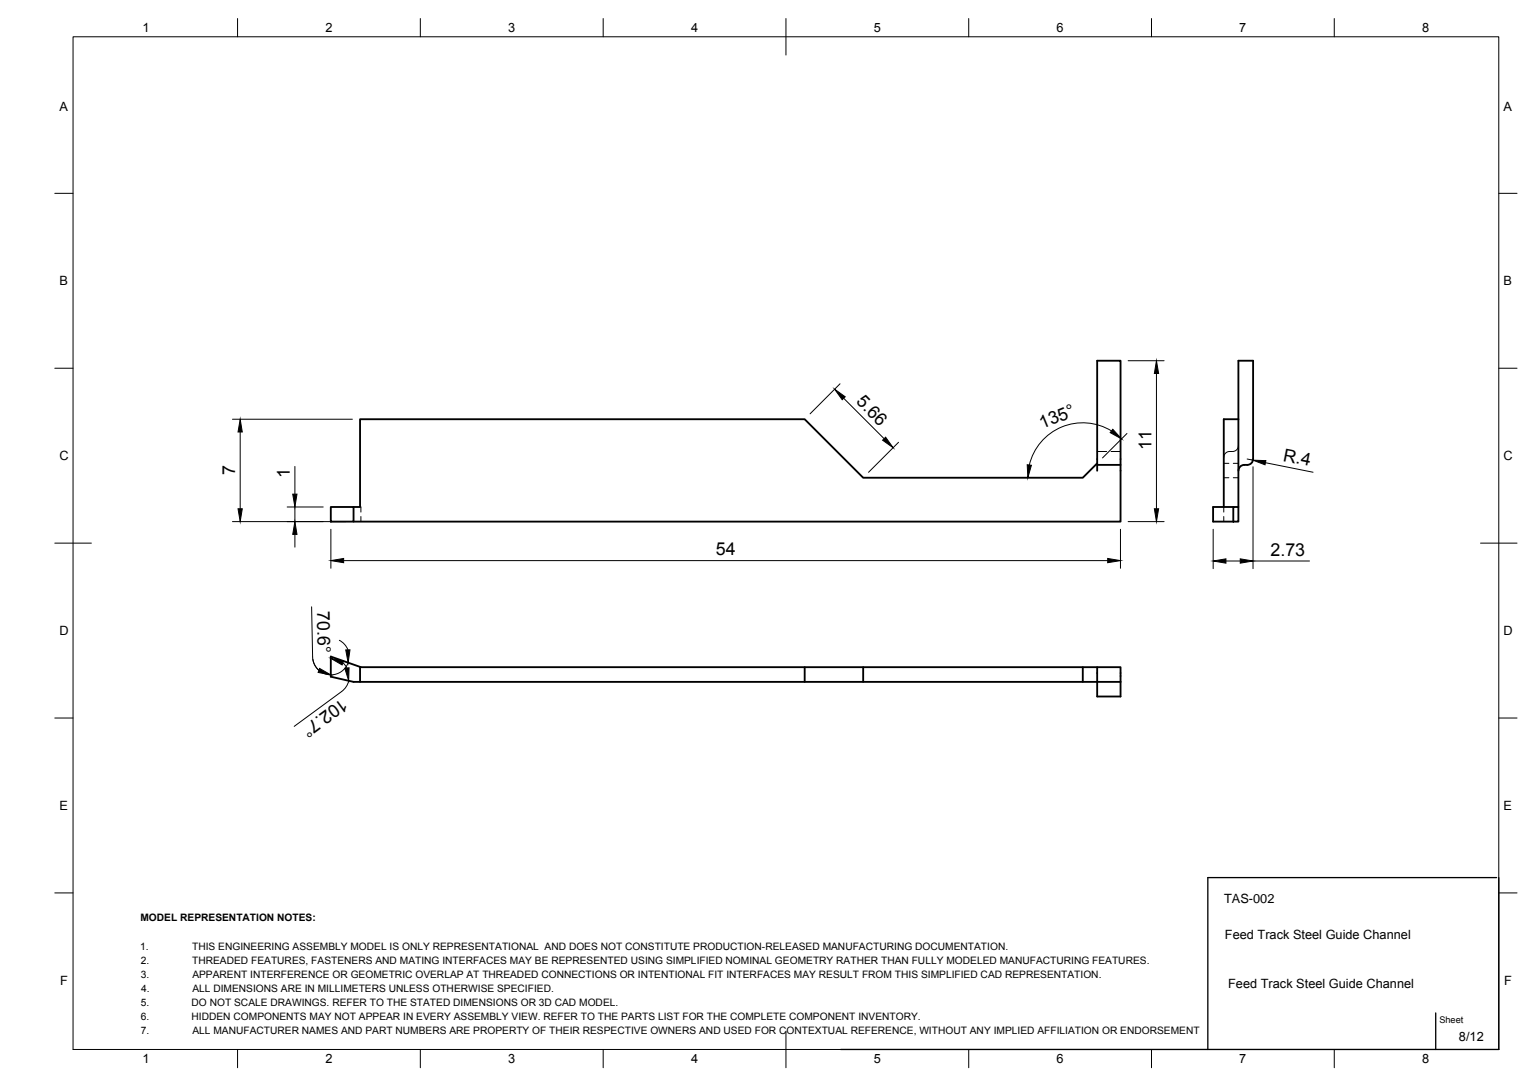
ISO-10303-21;
HEADER;
/* Generated by software containing ST-Developer
 * from STEP Tools, Inc. (www.steptools.com) 
 */

FILE_DESCRIPTION(
/* description */ ('STEP AP214'),
/* implementation_level */ '2;1');

FILE_NAME(
/* name */ 'Feed Track Steel Guide Channel.step',
/* time_stamp */ '2026-11-04T19:38:14-08:00',
/* author */ (''),
/* organization */ (''),
/* preprocessor_version */ 'ST-DEVELOPER v20.2',
/* originating_system */ 'Autodesk Translation Framework v15.17.0.0',
/* authorisation */ '');

FILE_SCHEMA (('AUTOMOTIVE_DESIGN { 1 0 10303 214 3 1 1 }'));
ENDSEC;

DATA;
#10=MECHANICAL_DESIGN_GEOMETRIC_PRESENTATION_REPRESENTATION('',(#475),#36668);
#455=SHAPE_REPRESENTATION_RELATIONSHIP('SRR','None',#36711,#465);
#465=ADVANCED_BREP_SHAPE_REPRESENTATION('',(#485),#36663);
#475=STYLED_ITEM('',(#36770),#485);
#485=MANIFOLD_SOLID_BREP('Body1',#17798);
#618=CYLINDRICAL_SURFACE('',#18758,0.399999999999998);
#619=CYLINDRICAL_SURFACE('',#18761,0.399999999999998);
#620=CYLINDRICAL_SURFACE('',#18764,0.399999999999998);
#621=CYLINDRICAL_SURFACE('',#18767,0.399999999999998);
#1353=CIRCLE('',#18759,0.399999999999998);
#1354=CIRCLE('',#18760,0.400000000000011);
#1355=CIRCLE('',#18762,0.399999999999998);
#1356=CIRCLE('',#18763,0.400000000000011);
#1357=CIRCLE('',#18765,0.400000000000011);
#1358=CIRCLE('',#18766,0.399999999999998);
#1359=CIRCLE('',#18768,0.400000000000011);
#1360=CIRCLE('',#18769,0.399999999999998);
#1973=FACE_OUTER_BOUND('',#3055,.T.);
#1974=FACE_OUTER_BOUND('',#3056,.T.);
#1975=FACE_OUTER_BOUND('',#3057,.T.);
#1976=FACE_OUTER_BOUND('',#3058,.T.);
#1977=FACE_OUTER_BOUND('',#3059,.T.);
#1978=FACE_OUTER_BOUND('',#3060,.T.);
#1979=FACE_OUTER_BOUND('',#3061,.T.);
#1980=FACE_OUTER_BOUND('',#3062,.T.);
#1981=FACE_OUTER_BOUND('',#3063,.T.);
#1982=FACE_OUTER_BOUND('',#3064,.T.);
#1983=FACE_OUTER_BOUND('',#3065,.T.);
#1984=FACE_OUTER_BOUND('',#3066,.T.);
#1985=FACE_OUTER_BOUND('',#3067,.T.);
#1986=FACE_OUTER_BOUND('',#3068,.T.);
#1987=FACE_OUTER_BOUND('',#3069,.T.);
#1988=FACE_OUTER_BOUND('',#3070,.T.);
#1989=FACE_OUTER_BOUND('',#3071,.T.);
#1990=FACE_OUTER_BOUND('',#3072,.T.);
#1991=FACE_OUTER_BOUND('',#3073,.T.);
#1992=FACE_OUTER_BOUND('',#3074,.T.);
#1993=FACE_OUTER_BOUND('',#3075,.T.);
#1994=FACE_OUTER_BOUND('',#3076,.T.);
#1995=FACE_OUTER_BOUND('',#3077,.T.);
#3055=EDGE_LOOP('',(#13714,#13715,#13716,#13717));
#3056=EDGE_LOOP('',(#13718,#13719,#13720,#13721));
#3057=EDGE_LOOP('',(#13722,#13723,#13724,#13725));
#3058=EDGE_LOOP('',(#13726,#13727,#13728,#13729));
#3059=EDGE_LOOP('',(#13730,#13731,#13732,#13733));
#3060=EDGE_LOOP('',(#13734,#13735,#13736,#13737));
#3061=EDGE_LOOP('',(#13738,#13739,#13740,#13741));
#3062=EDGE_LOOP('',(#13742,#13743,#13744,#13745));
#3063=EDGE_LOOP('',(#13746,#13747,#13748,#13749));
#3064=EDGE_LOOP('',(#13750,#13751,#13752,#13753));
#3065=EDGE_LOOP('',(#13754,#13755,#13756,#13757,#13758,#13759,#13760,#13761,
#13762,#13763,#13764));
#3066=EDGE_LOOP('',(#13765,#13766,#13767,#13768,#13769,#13770,#13771,#13772,
#13773,#13774,#13775));
#3067=EDGE_LOOP('',(#13776,#13777,#13778,#13779,#13780,#13781,#13782,#13783,
#13784,#13785,#13786,#13787));
#3068=EDGE_LOOP('',(#13788,#13789,#13790,#13791));
#3069=EDGE_LOOP('',(#13792,#13793,#13794,#13795));
#3070=EDGE_LOOP('',(#13796,#13797,#13798,#13799));
#3071=EDGE_LOOP('',(#13800,#13801,#13802,#13803));
#3072=EDGE_LOOP('',(#13804,#13805,#13806,#13807));
#3073=EDGE_LOOP('',(#13808,#13809,#13810,#13811,#13812,#13813));
#3074=EDGE_LOOP('',(#13814,#13815,#13816,#13817));
#3075=EDGE_LOOP('',(#13818,#13819,#13820,#13821,#13822,#13823,#13824,#13825,
#13826,#13827,#13828,#13829));
#3076=EDGE_LOOP('',(#13830,#13831,#13832,#13833));
#3077=EDGE_LOOP('',(#13834,#13835,#13836,#13837,#13838,#13839));
#4394=LINE('',#27429,#6104);
#4395=LINE('',#27431,#6105);
#4396=LINE('',#27433,#6106);
#4397=LINE('',#27434,#6107);
#4398=LINE('',#27438,#6108);
#4399=LINE('',#27440,#6109);
#4400=LINE('',#27442,#6110);
#4401=LINE('',#27443,#6111);
#4402=LINE('',#27449,#6112);
#4403=LINE('',#27452,#6113);
#4404=LINE('',#27458,#6114);
#4405=LINE('',#27461,#6115);
#4406=LINE('',#27467,#6116);
#4407=LINE('',#27470,#6117);
#4408=LINE('',#27476,#6118);
#4409=LINE('',#27479,#6119);
#4410=LINE('',#27482,#6120);
#4411=LINE('',#27484,#6121);
#4412=LINE('',#27485,#6122);
#4413=LINE('',#27487,#6123);
#4414=LINE('',#27488,#6124);
#4415=LINE('',#27491,#6125);
#4416=LINE('',#27493,#6126);
#4417=LINE('',#27494,#6127);
#4418=LINE('',#27496,#6128);
#4419=LINE('',#27497,#6129);
#4420=LINE('',#27500,#6130);
#4421=LINE('',#27501,#6131);
#4422=LINE('',#27503,#6132);
#4423=LINE('',#27505,#6133);
#4424=LINE('',#27507,#6134);
#4425=LINE('',#27509,#6135);
#4426=LINE('',#27511,#6136);
#4427=LINE('',#27513,#6137);
#4428=LINE('',#27514,#6138);
#4429=LINE('',#27517,#6139);
#4430=LINE('',#27518,#6140);
#4431=LINE('',#27520,#6141);
#4432=LINE('',#27522,#6142);
#4433=LINE('',#27524,#6143);
#4434=LINE('',#27526,#6144);
#4435=LINE('',#27528,#6145);
#4436=LINE('',#27530,#6146);
#4437=LINE('',#27531,#6147);
#4438=LINE('',#27533,#6148);
#4439=LINE('',#27534,#6149);
#4440=LINE('',#27536,#6150);
#4441=LINE('',#27538,#6151);
#4442=LINE('',#27540,#6152);
#4443=LINE('',#27542,#6153);
#4444=LINE('',#27544,#6154);
#4445=LINE('',#27546,#6155);
#4446=LINE('',#27548,#6156);
#4447=LINE('',#27550,#6157);
#4448=LINE('',#27551,#6158);
#6104=VECTOR('',#21930,1000.);
#6105=VECTOR('',#21931,1000.);
#6106=VECTOR('',#21932,1000.);
#6107=VECTOR('',#21933,1000.);
#6108=VECTOR('',#21936,1000.);
#6109=VECTOR('',#21937,1000.);
#6110=VECTOR('',#21938,1000.);
#6111=VECTOR('',#21939,1000.);
#6112=VECTOR('',#21944,1000.);
#6113=VECTOR('',#21947,1000.);
#6114=VECTOR('',#21952,1000.);
#6115=VECTOR('',#21955,1000.);
#6116=VECTOR('',#21960,1000.);
#6117=VECTOR('',#21963,1000.);
#6118=VECTOR('',#21968,1000.);
#6119=VECTOR('',#21971,1000.);
#6120=VECTOR('',#21974,1000.);
#6121=VECTOR('',#21975,1000.);
#6122=VECTOR('',#21976,1000.);
#6123=VECTOR('',#21979,1000.);
#6124=VECTOR('',#21980,1000.);
#6125=VECTOR('',#21983,1000.);
#6126=VECTOR('',#21984,1000.);
#6127=VECTOR('',#21985,1000.);
#6128=VECTOR('',#21988,1000.);
#6129=VECTOR('',#21989,1000.);
#6130=VECTOR('',#21992,1000.);
#6131=VECTOR('',#21993,1000.);
#6132=VECTOR('',#21994,1000.);
#6133=VECTOR('',#21995,1000.);
#6134=VECTOR('',#21996,1000.);
#6135=VECTOR('',#21997,1000.);
#6136=VECTOR('',#21998,1000.);
#6137=VECTOR('',#21999,1000.);
#6138=VECTOR('',#22000,1000.);
#6139=VECTOR('',#22003,1000.);
#6140=VECTOR('',#22004,1000.);
#6141=VECTOR('',#22005,1000.);
#6142=VECTOR('',#22006,1000.);
#6143=VECTOR('',#22007,1000.);
#6144=VECTOR('',#22008,1000.);
#6145=VECTOR('',#22009,1000.);
#6146=VECTOR('',#22010,1000.);
#6147=VECTOR('',#22011,1000.);
#6148=VECTOR('',#22014,1000.);
#6149=VECTOR('',#22015,1000.);
#6150=VECTOR('',#22018,1000.);
#6151=VECTOR('',#22021,1000.);
#6152=VECTOR('',#22024,1000.);
#6153=VECTOR('',#22027,1000.);
#6154=VECTOR('',#22030,1000.);
#6155=VECTOR('',#22033,1000.);
#6156=VECTOR('',#22036,1000.);
#6157=VECTOR('',#22039,1000.);
#6158=VECTOR('',#22040,1000.);
#7807=VERTEX_POINT('',#27427);
#7808=VERTEX_POINT('',#27428);
#7809=VERTEX_POINT('',#27430);
#7810=VERTEX_POINT('',#27432);
#7811=VERTEX_POINT('',#27436);
#7812=VERTEX_POINT('',#27437);
#7813=VERTEX_POINT('',#27439);
#7814=VERTEX_POINT('',#27441);
#7815=VERTEX_POINT('',#27445);
#7816=VERTEX_POINT('',#27446);
#7817=VERTEX_POINT('',#27448);
#7818=VERTEX_POINT('',#27450);
#7819=VERTEX_POINT('',#27454);
#7820=VERTEX_POINT('',#27455);
#7821=VERTEX_POINT('',#27457);
#7822=VERTEX_POINT('',#27459);
#7823=VERTEX_POINT('',#27463);
#7824=VERTEX_POINT('',#27464);
#7825=VERTEX_POINT('',#27466);
#7826=VERTEX_POINT('',#27468);
#7827=VERTEX_POINT('',#27472);
#7828=VERTEX_POINT('',#27473);
#7829=VERTEX_POINT('',#27475);
#7830=VERTEX_POINT('',#27477);
#7831=VERTEX_POINT('',#27481);
#7832=VERTEX_POINT('',#27483);
#7833=VERTEX_POINT('',#27490);
#7834=VERTEX_POINT('',#27492);
#7835=VERTEX_POINT('',#27499);
#7836=VERTEX_POINT('',#27502);
#7837=VERTEX_POINT('',#27504);
#7838=VERTEX_POINT('',#27506);
#7839=VERTEX_POINT('',#27508);
#7840=VERTEX_POINT('',#27510);
#7841=VERTEX_POINT('',#27512);
#7842=VERTEX_POINT('',#27516);
#7843=VERTEX_POINT('',#27519);
#7844=VERTEX_POINT('',#27521);
#7845=VERTEX_POINT('',#27523);
#7846=VERTEX_POINT('',#27525);
#7847=VERTEX_POINT('',#27527);
#7848=VERTEX_POINT('',#27529);
#9909=EDGE_CURVE('',#7807,#7808,#4394,.T.);
#9910=EDGE_CURVE('',#7809,#7807,#4395,.T.);
#9911=EDGE_CURVE('',#7809,#7810,#4396,.T.);
#9912=EDGE_CURVE('',#7810,#7808,#4397,.T.);
#9913=EDGE_CURVE('',#7811,#7812,#4398,.T.);
#9914=EDGE_CURVE('',#7813,#7812,#4399,.T.);
#9915=EDGE_CURVE('',#7814,#7813,#4400,.T.);
#9916=EDGE_CURVE('',#7814,#7811,#4401,.T.);
#9917=EDGE_CURVE('',#7815,#7816,#1353,.T.);
#9918=EDGE_CURVE('',#7817,#7815,#4402,.T.);
#9919=EDGE_CURVE('',#7818,#7817,#1354,.T.);
#9920=EDGE_CURVE('',#7816,#7818,#4403,.T.);
#9921=EDGE_CURVE('',#7819,#7820,#1355,.T.);
#9922=EDGE_CURVE('',#7821,#7819,#4404,.T.);
#9923=EDGE_CURVE('',#7822,#7821,#1356,.T.);
#9924=EDGE_CURVE('',#7820,#7822,#4405,.T.);
#9925=EDGE_CURVE('',#7823,#7824,#1357,.T.);
#9926=EDGE_CURVE('',#7825,#7823,#4406,.T.);
#9927=EDGE_CURVE('',#7826,#7825,#1358,.T.);
#9928=EDGE_CURVE('',#7824,#7826,#4407,.T.);
#9929=EDGE_CURVE('',#7827,#7828,#1359,.T.);
#9930=EDGE_CURVE('',#7829,#7827,#4408,.T.);
#9931=EDGE_CURVE('',#7830,#7829,#1360,.T.);
#9932=EDGE_CURVE('',#7828,#7830,#4409,.T.);
#9933=EDGE_CURVE('',#7831,#7820,#4410,.T.);
#9934=EDGE_CURVE('',#7822,#7832,#4411,.T.);
#9935=EDGE_CURVE('',#7832,#7831,#4412,.T.);
#9936=EDGE_CURVE('',#7821,#7818,#4413,.T.);
#9937=EDGE_CURVE('',#7819,#7816,#4414,.T.);
#9938=EDGE_CURVE('',#7833,#7824,#4415,.T.);
#9939=EDGE_CURVE('',#7826,#7834,#4416,.T.);
#9940=EDGE_CURVE('',#7834,#7833,#4417,.T.);
#9941=EDGE_CURVE('',#7823,#7828,#4418,.T.);
#9942=EDGE_CURVE('',#7825,#7830,#4419,.T.);
#9943=EDGE_CURVE('',#7835,#7812,#4420,.T.);
#9944=EDGE_CURVE('',#7829,#7835,#4421,.T.);
#9945=EDGE_CURVE('',#7836,#7827,#4422,.T.);
#9946=EDGE_CURVE('',#7837,#7836,#4423,.T.);
#9947=EDGE_CURVE('',#7838,#7837,#4424,.T.);
#9948=EDGE_CURVE('',#7839,#7838,#4425,.T.);
#9949=EDGE_CURVE('',#7840,#7839,#4426,.T.);
#9950=EDGE_CURVE('',#7841,#7840,#4427,.T.);
#9951=EDGE_CURVE('',#7813,#7841,#4428,.T.);
#9952=EDGE_CURVE('',#7815,#7842,#4429,.T.);
#9953=EDGE_CURVE('',#7842,#7808,#4430,.T.);
#9954=EDGE_CURVE('',#7810,#7843,#4431,.T.);
#9955=EDGE_CURVE('',#7843,#7844,#4432,.T.);
#9956=EDGE_CURVE('',#7844,#7845,#4433,.T.);
#9957=EDGE_CURVE('',#7845,#7846,#4434,.T.);
#9958=EDGE_CURVE('',#7846,#7847,#4435,.T.);
#9959=EDGE_CURVE('',#7847,#7848,#4436,.T.);
#9960=EDGE_CURVE('',#7848,#7817,#4437,.T.);
#9961=EDGE_CURVE('',#7832,#7833,#4438,.T.);
#9962=EDGE_CURVE('',#7848,#7836,#4439,.T.);
#9963=EDGE_CURVE('',#7847,#7837,#4440,.T.);
#9964=EDGE_CURVE('',#7846,#7838,#4441,.T.);
#9965=EDGE_CURVE('',#7845,#7839,#4442,.T.);
#9966=EDGE_CURVE('',#7844,#7840,#4443,.T.);
#9967=EDGE_CURVE('',#7843,#7841,#4444,.T.);
#9968=EDGE_CURVE('',#7809,#7814,#4445,.T.);
#9969=EDGE_CURVE('',#7807,#7811,#4446,.T.);
#9970=EDGE_CURVE('',#7842,#7835,#4447,.T.);
#9971=EDGE_CURVE('',#7831,#7834,#4448,.T.);
#13714=ORIENTED_EDGE('',*,*,#9909,.F.);
#13715=ORIENTED_EDGE('',*,*,#9910,.F.);
#13716=ORIENTED_EDGE('',*,*,#9911,.T.);
#13717=ORIENTED_EDGE('',*,*,#9912,.T.);
#13718=ORIENTED_EDGE('',*,*,#9913,.T.);
#13719=ORIENTED_EDGE('',*,*,#9914,.F.);
#13720=ORIENTED_EDGE('',*,*,#9915,.F.);
#13721=ORIENTED_EDGE('',*,*,#9916,.T.);
#13722=ORIENTED_EDGE('',*,*,#9917,.F.);
#13723=ORIENTED_EDGE('',*,*,#9918,.F.);
#13724=ORIENTED_EDGE('',*,*,#9919,.F.);
#13725=ORIENTED_EDGE('',*,*,#9920,.F.);
#13726=ORIENTED_EDGE('',*,*,#9921,.F.);
#13727=ORIENTED_EDGE('',*,*,#9922,.F.);
#13728=ORIENTED_EDGE('',*,*,#9923,.F.);
#13729=ORIENTED_EDGE('',*,*,#9924,.F.);
#13730=ORIENTED_EDGE('',*,*,#9925,.F.);
#13731=ORIENTED_EDGE('',*,*,#9926,.F.);
#13732=ORIENTED_EDGE('',*,*,#9927,.F.);
#13733=ORIENTED_EDGE('',*,*,#9928,.F.);
#13734=ORIENTED_EDGE('',*,*,#9929,.F.);
#13735=ORIENTED_EDGE('',*,*,#9930,.F.);
#13736=ORIENTED_EDGE('',*,*,#9931,.F.);
#13737=ORIENTED_EDGE('',*,*,#9932,.F.);
#13738=ORIENTED_EDGE('',*,*,#9933,.T.);
#13739=ORIENTED_EDGE('',*,*,#9924,.T.);
#13740=ORIENTED_EDGE('',*,*,#9934,.T.);
#13741=ORIENTED_EDGE('',*,*,#9935,.T.);
#13742=ORIENTED_EDGE('',*,*,#9936,.F.);
#13743=ORIENTED_EDGE('',*,*,#9922,.T.);
#13744=ORIENTED_EDGE('',*,*,#9937,.T.);
#13745=ORIENTED_EDGE('',*,*,#9920,.T.);
#13746=ORIENTED_EDGE('',*,*,#9938,.T.);
#13747=ORIENTED_EDGE('',*,*,#9928,.T.);
#13748=ORIENTED_EDGE('',*,*,#9939,.T.);
#13749=ORIENTED_EDGE('',*,*,#9940,.T.);
#13750=ORIENTED_EDGE('',*,*,#9941,.T.);
#13751=ORIENTED_EDGE('',*,*,#9932,.T.);
#13752=ORIENTED_EDGE('',*,*,#9942,.F.);
#13753=ORIENTED_EDGE('',*,*,#9926,.T.);
#13754=ORIENTED_EDGE('',*,*,#9943,.F.);
#13755=ORIENTED_EDGE('',*,*,#9944,.F.);
#13756=ORIENTED_EDGE('',*,*,#9930,.T.);
#13757=ORIENTED_EDGE('',*,*,#9945,.F.);
#13758=ORIENTED_EDGE('',*,*,#9946,.F.);
#13759=ORIENTED_EDGE('',*,*,#9947,.F.);
#13760=ORIENTED_EDGE('',*,*,#9948,.F.);
#13761=ORIENTED_EDGE('',*,*,#9949,.F.);
#13762=ORIENTED_EDGE('',*,*,#9950,.F.);
#13763=ORIENTED_EDGE('',*,*,#9951,.F.);
#13764=ORIENTED_EDGE('',*,*,#9914,.T.);
#13765=ORIENTED_EDGE('',*,*,#9952,.T.);
#13766=ORIENTED_EDGE('',*,*,#9953,.T.);
#13767=ORIENTED_EDGE('',*,*,#9912,.F.);
#13768=ORIENTED_EDGE('',*,*,#9954,.T.);
#13769=ORIENTED_EDGE('',*,*,#9955,.T.);
#13770=ORIENTED_EDGE('',*,*,#9956,.T.);
#13771=ORIENTED_EDGE('',*,*,#9957,.T.);
#13772=ORIENTED_EDGE('',*,*,#9958,.T.);
#13773=ORIENTED_EDGE('',*,*,#9959,.T.);
#13774=ORIENTED_EDGE('',*,*,#9960,.T.);
#13775=ORIENTED_EDGE('',*,*,#9918,.T.);
#13776=ORIENTED_EDGE('',*,*,#9941,.F.);
#13777=ORIENTED_EDGE('',*,*,#9925,.T.);
#13778=ORIENTED_EDGE('',*,*,#9938,.F.);
#13779=ORIENTED_EDGE('',*,*,#9961,.F.);
#13780=ORIENTED_EDGE('',*,*,#9934,.F.);
#13781=ORIENTED_EDGE('',*,*,#9923,.T.);
#13782=ORIENTED_EDGE('',*,*,#9936,.T.);
#13783=ORIENTED_EDGE('',*,*,#9919,.T.);
#13784=ORIENTED_EDGE('',*,*,#9960,.F.);
#13785=ORIENTED_EDGE('',*,*,#9962,.T.);
#13786=ORIENTED_EDGE('',*,*,#9945,.T.);
#13787=ORIENTED_EDGE('',*,*,#9929,.T.);
#13788=ORIENTED_EDGE('',*,*,#9946,.T.);
#13789=ORIENTED_EDGE('',*,*,#9962,.F.);
#13790=ORIENTED_EDGE('',*,*,#9959,.F.);
#13791=ORIENTED_EDGE('',*,*,#9963,.T.);
#13792=ORIENTED_EDGE('',*,*,#9947,.T.);
#13793=ORIENTED_EDGE('',*,*,#9963,.F.);
#13794=ORIENTED_EDGE('',*,*,#9958,.F.);
#13795=ORIENTED_EDGE('',*,*,#9964,.T.);
#13796=ORIENTED_EDGE('',*,*,#9948,.T.);
#13797=ORIENTED_EDGE('',*,*,#9964,.F.);
#13798=ORIENTED_EDGE('',*,*,#9957,.F.);
#13799=ORIENTED_EDGE('',*,*,#9965,.T.);
#13800=ORIENTED_EDGE('',*,*,#9949,.T.);
#13801=ORIENTED_EDGE('',*,*,#9965,.F.);
#13802=ORIENTED_EDGE('',*,*,#9956,.F.);
#13803=ORIENTED_EDGE('',*,*,#9966,.T.);
#13804=ORIENTED_EDGE('',*,*,#9950,.T.);
#13805=ORIENTED_EDGE('',*,*,#9966,.F.);
#13806=ORIENTED_EDGE('',*,*,#9955,.F.);
#13807=ORIENTED_EDGE('',*,*,#9967,.T.);
#13808=ORIENTED_EDGE('',*,*,#9968,.T.);
#13809=ORIENTED_EDGE('',*,*,#9915,.T.);
#13810=ORIENTED_EDGE('',*,*,#9951,.T.);
#13811=ORIENTED_EDGE('',*,*,#9967,.F.);
#13812=ORIENTED_EDGE('',*,*,#9954,.F.);
#13813=ORIENTED_EDGE('',*,*,#9911,.F.);
#13814=ORIENTED_EDGE('',*,*,#9969,.T.);
#13815=ORIENTED_EDGE('',*,*,#9916,.F.);
#13816=ORIENTED_EDGE('',*,*,#9968,.F.);
#13817=ORIENTED_EDGE('',*,*,#9910,.T.);
#13818=ORIENTED_EDGE('',*,*,#9939,.F.);
#13819=ORIENTED_EDGE('',*,*,#9927,.T.);
#13820=ORIENTED_EDGE('',*,*,#9942,.T.);
#13821=ORIENTED_EDGE('',*,*,#9931,.T.);
#13822=ORIENTED_EDGE('',*,*,#9944,.T.);
#13823=ORIENTED_EDGE('',*,*,#9970,.F.);
#13824=ORIENTED_EDGE('',*,*,#9952,.F.);
#13825=ORIENTED_EDGE('',*,*,#9917,.T.);
#13826=ORIENTED_EDGE('',*,*,#9937,.F.);
#13827=ORIENTED_EDGE('',*,*,#9921,.T.);
#13828=ORIENTED_EDGE('',*,*,#9933,.F.);
#13829=ORIENTED_EDGE('',*,*,#9971,.T.);
#13830=ORIENTED_EDGE('',*,*,#9935,.F.);
#13831=ORIENTED_EDGE('',*,*,#9961,.T.);
#13832=ORIENTED_EDGE('',*,*,#9940,.F.);
#13833=ORIENTED_EDGE('',*,*,#9971,.F.);
#13834=ORIENTED_EDGE('',*,*,#9943,.T.);
#13835=ORIENTED_EDGE('',*,*,#9913,.F.);
#13836=ORIENTED_EDGE('',*,*,#9969,.F.);
#13837=ORIENTED_EDGE('',*,*,#9909,.T.);
#13838=ORIENTED_EDGE('',*,*,#9953,.F.);
#13839=ORIENTED_EDGE('',*,*,#9970,.T.);
#16565=PLANE('',#18756);
#16566=PLANE('',#18757);
#16567=PLANE('',#18770);
#16568=PLANE('',#18771);
#16569=PLANE('',#18772);
#16570=PLANE('',#18773);
#16571=PLANE('',#18774);
#16572=PLANE('',#18775);
#16573=PLANE('',#18776);
#16574=PLANE('',#18777);
#16575=PLANE('',#18778);
#16576=PLANE('',#18779);
#16577=PLANE('',#18780);
#16578=PLANE('',#18781);
#16579=PLANE('',#18782);
#16580=PLANE('',#18783);
#16581=PLANE('',#18784);
#16582=PLANE('',#18785);
#16583=PLANE('',#18786);
#17308=ADVANCED_FACE('',(#1973),#16565,.T.);
#17309=ADVANCED_FACE('',(#1974),#16566,.F.);
#17310=ADVANCED_FACE('',(#1975),#618,.T.);
#17311=ADVANCED_FACE('',(#1976),#619,.F.);
#17312=ADVANCED_FACE('',(#1977),#620,.T.);
#17313=ADVANCED_FACE('',(#1978),#621,.F.);
#17314=ADVANCED_FACE('',(#1979),#16567,.T.);
#17315=ADVANCED_FACE('',(#1980),#16568,.F.);
#17316=ADVANCED_FACE('',(#1981),#16569,.T.);
#17317=ADVANCED_FACE('',(#1982),#16570,.F.);
#17318=ADVANCED_FACE('',(#1983),#16571,.T.);
#17319=ADVANCED_FACE('',(#1984),#16572,.F.);
#17320=ADVANCED_FACE('',(#1985),#16573,.F.);
#17321=ADVANCED_FACE('',(#1986),#16574,.F.);
#17322=ADVANCED_FACE('',(#1987),#16575,.F.);
#17323=ADVANCED_FACE('',(#1988),#16576,.F.);
#17324=ADVANCED_FACE('',(#1989),#16577,.F.);
#17325=ADVANCED_FACE('',(#1990),#16578,.F.);
#17326=ADVANCED_FACE('',(#1991),#16579,.F.);
#17327=ADVANCED_FACE('',(#1992),#16580,.F.);
#17328=ADVANCED_FACE('',(#1993),#16581,.F.);
#17329=ADVANCED_FACE('',(#1994),#16582,.F.);
#17330=ADVANCED_FACE('',(#1995),#16583,.F.);
#17798=CLOSED_SHELL('',(#17308,#17309,#17310,#17311,#17312,#17313,#17314,
#17315,#17316,#17317,#17318,#17319,#17320,#17321,#17322,#17323,#17324,#17325,
#17326,#17327,#17328,#17329,#17330));
#18755=AXIS2_PLACEMENT_3D('',#27425,#21926,#21927);
#18756=AXIS2_PLACEMENT_3D('',#27426,#21928,#21929);
#18757=AXIS2_PLACEMENT_3D('',#27435,#21934,#21935);
#18758=AXIS2_PLACEMENT_3D('',#27444,#21940,#21941);
#18759=AXIS2_PLACEMENT_3D('',#27447,#21942,#21943);
#18760=AXIS2_PLACEMENT_3D('',#27451,#21945,#21946);
#18761=AXIS2_PLACEMENT_3D('',#27453,#21948,#21949);
#18762=AXIS2_PLACEMENT_3D('',#27456,#21950,#21951);
#18763=AXIS2_PLACEMENT_3D('',#27460,#21953,#21954);
#18764=AXIS2_PLACEMENT_3D('',#27462,#21956,#21957);
#18765=AXIS2_PLACEMENT_3D('',#27465,#21958,#21959);
#18766=AXIS2_PLACEMENT_3D('',#27469,#21961,#21962);
#18767=AXIS2_PLACEMENT_3D('',#27471,#21964,#21965);
#18768=AXIS2_PLACEMENT_3D('',#27474,#21966,#21967);
#18769=AXIS2_PLACEMENT_3D('',#27478,#21969,#21970);
#18770=AXIS2_PLACEMENT_3D('',#27480,#21972,#21973);
#18771=AXIS2_PLACEMENT_3D('',#27486,#21977,#21978);
#18772=AXIS2_PLACEMENT_3D('',#27489,#21981,#21982);
#18773=AXIS2_PLACEMENT_3D('',#27495,#21986,#21987);
#18774=AXIS2_PLACEMENT_3D('',#27498,#21990,#21991);
#18775=AXIS2_PLACEMENT_3D('',#27515,#22001,#22002);
#18776=AXIS2_PLACEMENT_3D('',#27532,#22012,#22013);
#18777=AXIS2_PLACEMENT_3D('',#27535,#22016,#22017);
#18778=AXIS2_PLACEMENT_3D('',#27537,#22019,#22020);
#18779=AXIS2_PLACEMENT_3D('',#27539,#22022,#22023);
#18780=AXIS2_PLACEMENT_3D('',#27541,#22025,#22026);
#18781=AXIS2_PLACEMENT_3D('',#27543,#22028,#22029);
#18782=AXIS2_PLACEMENT_3D('',#27545,#22031,#22032);
#18783=AXIS2_PLACEMENT_3D('',#27547,#22034,#22035);
#18784=AXIS2_PLACEMENT_3D('',#27549,#22037,#22038);
#18785=AXIS2_PLACEMENT_3D('',#27552,#22041,#22042);
#18786=AXIS2_PLACEMENT_3D('',#27553,#22043,#22044);
#21926=DIRECTION('axis',(0.,0.,1.));
#21927=DIRECTION('refdir',(1.,0.,0.));
#21928=DIRECTION('center_axis',(-0.332226829439148,0.943199519614387,0.));
#21929=DIRECTION('ref_axis',(0.,0.,-1.));
#21930=DIRECTION('',(-0.943199519614387,-0.332226829439149,0.));
#21931=DIRECTION('',(0.,0.,1.));
#21932=DIRECTION('',(-0.943199519614387,-0.332226829439149,0.));
#21933=DIRECTION('',(0.,0.,1.));
#21934=DIRECTION('center_axis',(-0.219923546994498,0.975517110807063,0.));
#21935=DIRECTION('ref_axis',(0.,0.,-1.));
#21936=DIRECTION('',(-0.975517110807063,-0.219923546994498,0.));
#21937=DIRECTION('',(0.,0.,1.));
#21938=DIRECTION('',(-0.975517110807063,-0.219923546994498,0.));
#21939=DIRECTION('',(0.,0.,1.));
#21940=DIRECTION('center_axis',(1.,-1.E-15,0.));
#21941=DIRECTION('ref_axis',(-1.E-15,-1.,0.));
#21942=DIRECTION('center_axis',(-1.,1.E-15,0.));
#21943=DIRECTION('ref_axis',(-1.E-15,-1.,0.));
#21944=DIRECTION('',(-1.,1.E-15,0.));
#21945=DIRECTION('center_axis',(1.,-1.E-15,0.));
#21946=DIRECTION('ref_axis',(0.,0.,1.));
#21947=DIRECTION('',(1.,-1.E-15,0.));
#21948=DIRECTION('center_axis',(1.,-1.E-15,0.));
#21949=DIRECTION('ref_axis',(-1.E-15,-1.,0.));
#21950=DIRECTION('center_axis',(1.,-1.E-15,0.));
#21951=DIRECTION('ref_axis',(-1.E-15,-1.,0.));
#21952=DIRECTION('',(-1.,1.E-15,0.));
#21953=DIRECTION('center_axis',(-1.,1.E-15,0.));
#21954=DIRECTION('ref_axis',(0.,0.,1.));
#21955=DIRECTION('',(1.,-1.E-15,0.));
#21956=DIRECTION('center_axis',(1.,-1.E-15,0.));
#21957=DIRECTION('ref_axis',(-1.E-15,-1.,0.));
#21958=DIRECTION('center_axis',(1.,-1.E-15,0.));
#21959=DIRECTION('ref_axis',(0.,0.,1.));
#21960=DIRECTION('',(1.,-1.E-15,0.));
#21961=DIRECTION('center_axis',(-1.,1.E-15,0.));
#21962=DIRECTION('ref_axis',(-1.E-15,-1.,0.));
#21963=DIRECTION('',(-1.,1.E-15,0.));
#21964=DIRECTION('center_axis',(-1.,1.E-15,0.));
#21965=DIRECTION('ref_axis',(1.E-15,1.,0.));
#21966=DIRECTION('center_axis',(-1.,1.E-15,0.));
#21967=DIRECTION('ref_axis',(0.,0.,1.));
#21968=DIRECTION('',(1.,-1.E-15,0.));
#21969=DIRECTION('center_axis',(1.,-1.E-15,0.));
#21970=DIRECTION('ref_axis',(-1.E-15,-1.,0.));
#21971=DIRECTION('',(-1.,1.E-15,0.));
#21972=DIRECTION('center_axis',(1.E-15,1.,0.));
#21973=DIRECTION('ref_axis',(1.,-1.E-15,0.));
#21974=DIRECTION('',(0.,0.,1.));
#21975=DIRECTION('',(0.,0.,-1.));
#21976=DIRECTION('',(-1.,1.E-15,0.));
#21977=DIRECTION('center_axis',(0.,0.,1.));
#21978=DIRECTION('ref_axis',(-1.E-15,-1.,0.));
#21979=DIRECTION('',(1.E-15,1.,0.));
#21980=DIRECTION('',(1.E-15,1.,0.));
#21981=DIRECTION('center_axis',(-1.E-15,-1.,0.));
#21982=DIRECTION('ref_axis',(0.,0.,1.));
#21983=DIRECTION('',(0.,0.,1.));
#21984=DIRECTION('',(0.,0.,-1.));
#21985=DIRECTION('',(1.,-1.E-15,0.));
#21986=DIRECTION('center_axis',(0.,0.,-1.));
#21987=DIRECTION('ref_axis',(1.,-1.E-15,0.));
#21988=DIRECTION('',(1.E-15,1.,0.));
#21989=DIRECTION('',(1.E-15,1.,0.));
#21990=DIRECTION('center_axis',(-1.E-15,-1.,0.));
#21991=DIRECTION('ref_axis',(0.,0.,1.));
#21992=DIRECTION('',(1.,-1.E-15,0.));
#21993=DIRECTION('',(0.,0.,1.));
#21994=DIRECTION('',(0.,0.,1.));
#21995=DIRECTION('',(-0.707106781186547,7.07106781186548E-16,-0.707106781186547));
#21996=DIRECTION('',(-1.,1.E-15,-5.77559370956749E-17));
#21997=DIRECTION('',(-0.707106781186547,7.07106781186547E-16,0.707106781186548));
#21998=DIRECTION('',(-1.,1.E-15,0.));
#21999=DIRECTION('',(0.,0.,-1.));
#22000=DIRECTION('',(-1.,1.E-15,0.));
#22001=DIRECTION('center_axis',(-1.E-15,-1.,0.));
#22002=DIRECTION('ref_axis',(0.,0.,1.));
#22003=DIRECTION('',(0.,0.,1.));
#22004=DIRECTION('',(1.,-1.E-15,0.));
#22005=DIRECTION('',(1.,-1.E-15,0.));
#22006=DIRECTION('',(0.,0.,-1.));
#22007=DIRECTION('',(-1.,1.E-15,0.));
#22008=DIRECTION('',(-0.707106781186547,7.07106781186547E-16,0.707106781186548));
#22009=DIRECTION('',(-1.,1.E-15,-5.77559370956749E-17));
#22010=DIRECTION('',(-0.707106781186547,7.07106781186548E-16,-0.707106781186547));
#22011=DIRECTION('',(4.94384700890794E-16,-4.94384700890794E-31,-1.));
#22012=DIRECTION('center_axis',(-1.,1.E-15,-4.94384700890794E-16));
#22013=DIRECTION('ref_axis',(1.E-15,1.,-2.03147768281658E-47));
#22014=DIRECTION('',(-1.E-15,-1.,0.));
#22015=DIRECTION('',(-1.E-15,-1.,0.));
#22016=DIRECTION('center_axis',(-0.707106781186548,7.07106781186548E-16,
0.707106781186548));
#22017=DIRECTION('ref_axis',(-0.707106781186548,7.07106781186547E-16,-0.707106781186548));
#22018=DIRECTION('',(-1.E-15,-1.,0.));
#22019=DIRECTION('center_axis',(-5.77559370956749E-17,5.77559370956749E-32,
1.));
#22020=DIRECTION('ref_axis',(-1.,1.E-15,-5.77559370956749E-17));
#22021=DIRECTION('',(-1.E-15,-1.,0.));
#22022=DIRECTION('center_axis',(0.707106781186548,-7.07106781186548E-16,
0.707106781186547));
#22023=DIRECTION('ref_axis',(-1.E-15,-1.,4.22628099173863E-32));
#22024=DIRECTION('',(-1.E-15,-1.,0.));
#22025=DIRECTION('center_axis',(0.,0.,1.));
#22026=DIRECTION('ref_axis',(-1.E-15,-1.,0.));
#22027=DIRECTION('',(-1.E-15,-1.,0.));
#22028=DIRECTION('center_axis',(-1.,1.E-15,0.));
#22029=DIRECTION('ref_axis',(1.E-15,1.,0.));
#22030=DIRECTION('',(-1.E-15,-1.,0.));
#22031=DIRECTION('center_axis',(0.,0.,1.));
#22032=DIRECTION('ref_axis',(-1.E-15,-1.,0.));
#22033=DIRECTION('',(-1.E-15,-1.,0.));
#22034=DIRECTION('center_axis',(-1.,1.E-15,6.93889390390723E-15));
#22035=DIRECTION('ref_axis',(-6.93889390390723E-15,6.93889390390723E-30,
-1.));
#22036=DIRECTION('',(-1.E-15,-1.,0.));
#22037=DIRECTION('center_axis',(1.,-1.E-15,0.));
#22038=DIRECTION('ref_axis',(0.,0.,-1.));
#22039=DIRECTION('',(-1.E-15,-1.,0.));
#22040=DIRECTION('',(-1.E-15,-1.,0.));
#22041=DIRECTION('center_axis',(0.,0.,1.));
#22042=DIRECTION('ref_axis',(-1.E-15,-1.,0.));
#22043=DIRECTION('center_axis',(0.,0.,-1.));
#22044=DIRECTION('ref_axis',(1.,-1.E-15,0.));
#27425=CARTESIAN_POINT('',(0.,0.,0.));
#27426=CARTESIAN_POINT('Origin',(-20.4739437433364,34.556757731995,212.621369141518));
#27427=CARTESIAN_POINT('',(-18.4141818172079,35.2822756737311,213.621369141518));
#27428=CARTESIAN_POINT('',(-20.4739437433364,34.556757731995,213.621369141518));
#27429=CARTESIAN_POINT('',(-20.4739437433364,34.556757731995,213.621369141518));
#27430=CARTESIAN_POINT('',(-18.4141818172079,35.2822756737311,212.621369141518));
#27431=CARTESIAN_POINT('',(-18.4141818172079,35.2822756737311,212.621369141518));
#27432=CARTESIAN_POINT('',(-20.4739437433364,34.556757731995,212.621369141518));
#27433=CARTESIAN_POINT('',(-20.4739437433364,34.556757731995,212.621369141518));
#27434=CARTESIAN_POINT('',(-20.4739437433364,34.556757731995,212.621369141518));
#27435=CARTESIAN_POINT('Origin',(-19.9693351501811,33.556757731995,212.621369141518));
#27436=CARTESIAN_POINT('',(-18.4141818172079,33.907356233363,213.621369141518));
#27437=CARTESIAN_POINT('',(-19.9693351501811,33.556757731995,213.621369141518));
#27438=CARTESIAN_POINT('',(-19.9693351501811,33.556757731995,213.621369141518));
#27439=CARTESIAN_POINT('',(-19.9693351501811,33.556757731995,212.621369141518));
#27440=CARTESIAN_POINT('',(-19.9693351501811,33.556757731995,212.621369141518));
#27441=CARTESIAN_POINT('',(-18.4141818172079,33.907356233363,212.621369141518));
#27442=CARTESIAN_POINT('',(-19.9693351501811,33.556757731995,212.621369141518));
#27443=CARTESIAN_POINT('',(-18.4141818172079,33.907356233363,212.621369141518));
#27444=CARTESIAN_POINT('Origin',(-70.8141818172079,34.156757731995,209.227232600396));
#27445=CARTESIAN_POINT('',(-72.4141818172079,34.556757731995,209.227232600396));
#27446=CARTESIAN_POINT('',(-72.4141818172079,34.156757731995,208.827232600396));
#27447=CARTESIAN_POINT('Origin',(-72.4141818172079,34.156757731995,209.227232600396));
#27448=CARTESIAN_POINT('',(-70.8141818172079,34.556757731995,209.227232600396));
#27449=CARTESIAN_POINT('',(-47.969665759339,34.556757731995,209.227232600396));
#27450=CARTESIAN_POINT('',(-70.8141818172079,34.156757731995,208.827232600396));
#27451=CARTESIAN_POINT('Origin',(-70.8141818172079,34.156757731995,209.227232600396));
#27452=CARTESIAN_POINT('',(-70.8141818172079,34.156757731995,208.827232600396));
#27453=CARTESIAN_POINT('Origin',(-47.969665759339,33.956757731995,208.427232600396));
#27454=CARTESIAN_POINT('',(-72.4141818172079,33.956757731995,208.827232600396));
#27455=CARTESIAN_POINT('',(-72.4141818172079,33.556757731995,208.427232600396));
#27456=CARTESIAN_POINT('Origin',(-72.4141818172079,33.956757731995,208.427232600396));
#27457=CARTESIAN_POINT('',(-70.8141818172079,33.956757731995,208.827232600396));
#27458=CARTESIAN_POINT('',(-70.8141818172079,33.956757731995,208.827232600396));
#27459=CARTESIAN_POINT('',(-70.8141818172079,33.556757731995,208.427232600396));
#27460=CARTESIAN_POINT('Origin',(-70.8141818172079,33.956757731995,208.427232600396));
#27461=CARTESIAN_POINT('',(-47.969665759339,33.556757731995,208.427232600396));
#27462=CARTESIAN_POINT('Origin',(-47.969665759339,32.956757731995,209.344010998233));
#27463=CARTESIAN_POINT('',(-70.8141818172079,32.956757731995,209.744010998233));
#27464=CARTESIAN_POINT('',(-70.8141818172079,32.556757731995,209.344010998233));
#27465=CARTESIAN_POINT('Origin',(-70.8141818172079,32.956757731995,209.344010998233));
#27466=CARTESIAN_POINT('',(-72.4141818172079,32.956757731995,209.744010998233));
#27467=CARTESIAN_POINT('',(-70.8141818172079,32.956757731995,209.744010998233));
#27468=CARTESIAN_POINT('',(-72.4141818172079,32.556757731995,209.344010998233));
#27469=CARTESIAN_POINT('Origin',(-72.4141818172079,32.956757731995,209.344010998233));
#27470=CARTESIAN_POINT('',(-72.4141818172079,32.556757731995,209.344010998233));
#27471=CARTESIAN_POINT('Origin',(-70.8141818172079,33.156757731995,210.144010998233));
#27472=CARTESIAN_POINT('',(-70.8141818172079,33.556757731995,210.144010998233));
#27473=CARTESIAN_POINT('',(-70.8141818172079,33.156757731995,209.744010998233));
#27474=CARTESIAN_POINT('Origin',(-70.8141818172079,33.156757731995,210.144010998233));
#27475=CARTESIAN_POINT('',(-72.4141818172079,33.556757731995,210.144010998233));
#27476=CARTESIAN_POINT('',(-47.969665759339,33.556757731995,210.144010998233));
#27477=CARTESIAN_POINT('',(-72.4141818172079,33.156757731995,209.744010998233));
#27478=CARTESIAN_POINT('Origin',(-72.4141818172079,33.156757731995,210.144010998233));
#27479=CARTESIAN_POINT('',(-70.8141818172079,33.156757731995,209.744010998233));
#27480=CARTESIAN_POINT('Origin',(-47.969665759339,33.556757731995,213.621369141518));
#27481=CARTESIAN_POINT('',(-72.4141818172079,33.556757731995,202.621369141518));
#27482=CARTESIAN_POINT('',(-72.4141818172079,33.556757731995,208.827232600396));
#27483=CARTESIAN_POINT('',(-70.8141818172079,33.556757731995,202.621369141518));
#27484=CARTESIAN_POINT('',(-70.8141818172079,33.556757731995,208.827232600396));
#27485=CARTESIAN_POINT('',(-70.8141818172079,33.556757731995,202.621369141518));
#27486=CARTESIAN_POINT('Origin',(-70.8141818172079,33.556757731995,208.827232600396));
#27487=CARTESIAN_POINT('',(-70.8141818172079,33.556757731995,208.827232600396));
#27488=CARTESIAN_POINT('',(-72.4141818172079,33.556757731995,208.827232600396));
#27489=CARTESIAN_POINT('Origin',(-47.969665759339,32.556757731995,213.621369141518));
#27490=CARTESIAN_POINT('',(-70.8141818172079,32.556757731995,202.621369141518));
#27491=CARTESIAN_POINT('',(-70.8141818172079,32.556757731995,202.621369141518));
#27492=CARTESIAN_POINT('',(-72.4141818172079,32.556757731995,202.621369141518));
#27493=CARTESIAN_POINT('',(-72.4141818172079,32.556757731995,202.621369141518));
#27494=CARTESIAN_POINT('',(-70.8141818172079,32.556757731995,202.621369141518));
#27495=CARTESIAN_POINT('Origin',(-70.8141818172079,32.556757731995,209.744010998233));
#27496=CARTESIAN_POINT('',(-70.8141818172079,32.556757731995,209.744010998233));
#27497=CARTESIAN_POINT('',(-72.4141818172079,32.556757731995,209.744010998233));
#27498=CARTESIAN_POINT('Origin',(-47.969665759339,33.556757731995,213.621369141518));
#27499=CARTESIAN_POINT('',(-72.4141818172079,33.556757731995,213.621369141518));
#27500=CARTESIAN_POINT('',(-72.4141818172079,33.556757731995,213.621369141518));
#27501=CARTESIAN_POINT('',(-72.4141818172079,33.556757731995,213.621369141518));
#27502=CARTESIAN_POINT('',(-70.8141818172079,33.556757731995,209.639076092608));
#27503=CARTESIAN_POINT('',(-70.8141818172079,33.556757731995,202.621369141518));
#27504=CARTESIAN_POINT('',(-69.8318887682974,33.556757731995,210.621369141518));
#27505=CARTESIAN_POINT('',(-70.8141818172079,33.556757731995,209.639076092608));
#27506=CARTESIAN_POINT('',(-54.8141818172079,33.556757731995,210.621369141518));
#27507=CARTESIAN_POINT('',(-69.8318887682974,33.556757731995,210.621369141518));
#27508=CARTESIAN_POINT('',(-50.8141818172079,33.556757731995,206.621369141518));
#27509=CARTESIAN_POINT('',(-54.8141818172079,33.556757731995,210.621369141518));
#27510=CARTESIAN_POINT('',(-20.4141818172079,33.556757731995,206.621369141518));
#27511=CARTESIAN_POINT('',(-50.8141818172079,33.556757731995,206.621369141518));
#27512=CARTESIAN_POINT('',(-20.4141818172079,33.556757731995,212.621369141518));
#27513=CARTESIAN_POINT('',(-20.4141818172079,33.556757731995,206.621369141518));
#27514=CARTESIAN_POINT('',(-20.4141818172079,33.556757731995,212.621369141518));
#27515=CARTESIAN_POINT('Origin',(-47.969665759339,34.556757731995,213.621369141518));
#27516=CARTESIAN_POINT('',(-72.4141818172079,34.556757731995,213.621369141518));
#27517=CARTESIAN_POINT('',(-72.4141818172079,34.556757731995,213.621369141518));
#27518=CARTESIAN_POINT('',(-72.4141818172079,34.556757731995,213.621369141518));
#27519=CARTESIAN_POINT('',(-20.4141818172079,34.556757731995,212.621369141518));
#27520=CARTESIAN_POINT('',(-18.4141818172079,34.556757731995,212.621369141518));
#27521=CARTESIAN_POINT('',(-20.4141818172079,34.556757731995,206.621369141518));
#27522=CARTESIAN_POINT('',(-20.4141818172079,34.556757731995,206.621369141518));
#27523=CARTESIAN_POINT('',(-50.8141818172079,34.556757731995,206.621369141518));
#27524=CARTESIAN_POINT('',(-50.8141818172079,34.556757731995,206.621369141518));
#27525=CARTESIAN_POINT('',(-54.8141818172079,34.556757731995,210.621369141518));
#27526=CARTESIAN_POINT('',(-54.8141818172079,34.556757731995,210.621369141518));
#27527=CARTESIAN_POINT('',(-69.8318887682974,34.556757731995,210.621369141518));
#27528=CARTESIAN_POINT('',(-69.8318887682974,34.556757731995,210.621369141518));
#27529=CARTESIAN_POINT('',(-70.8141818172079,34.556757731995,209.639076092608));
#27530=CARTESIAN_POINT('',(-70.8141818172079,34.556757731995,209.639076092608));
#27531=CARTESIAN_POINT('',(-70.8141818172079,34.556757731995,202.621369141518));
#27532=CARTESIAN_POINT('Origin',(-70.8141818172079,34.556757731995,202.621369141518));
#27533=CARTESIAN_POINT('',(-70.8141818172079,34.556757731995,202.621369141518));
#27534=CARTESIAN_POINT('',(-70.8141818172079,34.556757731995,209.639076092608));
#27535=CARTESIAN_POINT('Origin',(-70.8141818172079,34.556757731995,209.639076092608));
#27536=CARTESIAN_POINT('',(-69.8318887682974,34.556757731995,210.621369141518));
#27537=CARTESIAN_POINT('Origin',(-69.8318887682974,34.556757731995,210.621369141518));
#27538=CARTESIAN_POINT('',(-54.8141818172079,34.556757731995,210.621369141518));
#27539=CARTESIAN_POINT('Origin',(-54.8141818172079,34.556757731995,210.621369141518));
#27540=CARTESIAN_POINT('',(-50.8141818172079,34.556757731995,206.621369141518));
#27541=CARTESIAN_POINT('Origin',(-50.8141818172079,34.556757731995,206.621369141518));
#27542=CARTESIAN_POINT('',(-20.4141818172079,34.556757731995,206.621369141518));
#27543=CARTESIAN_POINT('Origin',(-20.4141818172079,34.556757731995,206.621369141518));
#27544=CARTESIAN_POINT('',(-20.4141818172079,34.556757731995,212.621369141518));
#27545=CARTESIAN_POINT('Origin',(-20.4141818172079,34.556757731995,212.621369141518));
#27546=CARTESIAN_POINT('',(-18.4141818172079,34.556757731995,212.621369141518));
#27547=CARTESIAN_POINT('Origin',(-18.4141818172079,34.556757731995,212.621369141518));
#27548=CARTESIAN_POINT('',(-18.4141818172079,34.556757731995,213.621369141518));
#27549=CARTESIAN_POINT('Origin',(-72.4141818172079,34.556757731995,213.621369141518));
#27550=CARTESIAN_POINT('',(-72.4141818172079,34.556757731995,213.621369141518));
#27551=CARTESIAN_POINT('',(-72.4141818172079,34.556757731995,202.621369141518));
#27552=CARTESIAN_POINT('Origin',(-72.4141818172079,34.556757731995,202.621369141518));
#27553=CARTESIAN_POINT('Origin',(-72.4141818172079,34.556757731995,213.621369141518));
#36651=UNCERTAINTY_MEASURE_WITH_UNIT(LENGTH_MEASURE(0.01),#36669,
'DISTANCE_ACCURACY_VALUE',
'Maximum model space distance between geometric entities at asserted c
onnectivities');
#36656=UNCERTAINTY_MEASURE_WITH_UNIT(LENGTH_MEASURE(0.01),#36669,
'DISTANCE_ACCURACY_VALUE',
'Maximum model space distance between geometric entities at asserted c
onnectivities');
#36663=(
GEOMETRIC_REPRESENTATION_CONTEXT(3)
GLOBAL_UNCERTAINTY_ASSIGNED_CONTEXT((#36651))
GLOBAL_UNIT_ASSIGNED_CONTEXT((#36669,#36671,#36672))
REPRESENTATION_CONTEXT('','3D')
);
#36668=(
GEOMETRIC_REPRESENTATION_CONTEXT(3)
GLOBAL_UNCERTAINTY_ASSIGNED_CONTEXT((#36656))
GLOBAL_UNIT_ASSIGNED_CONTEXT((#36669,#36671,#36672))
REPRESENTATION_CONTEXT('','3D')
);
#36669=(
LENGTH_UNIT()
NAMED_UNIT(*)
SI_UNIT(.MILLI.,.METRE.)
);
#36671=(
NAMED_UNIT(*)
PLANE_ANGLE_UNIT()
SI_UNIT($,.RADIAN.)
);
#36672=(
NAMED_UNIT(*)
SI_UNIT($,.STERADIAN.)
SOLID_ANGLE_UNIT()
);
#36679=SHAPE_DEFINITION_REPRESENTATION(#36690,#36711);
#36690=PRODUCT_DEFINITION_SHAPE('',$,#36723);
#36711=SHAPE_REPRESENTATION('',(#18755),#36663);
#36716=PRODUCT_DEFINITION_CONTEXT('part definition',#36751,'design');
#36723=PRODUCT_DEFINITION('Feed Track Steel Guide Channel',
'Feed Track Steel Guide Channel',#36734,#36716);
#36734=PRODUCT_DEFINITION_FORMATION('',$,#36759);
#36751=APPLICATION_CONTEXT(
'Core Data for Automotive Mechanical Design Process');
#36752=PRODUCT_CONTEXT('part definition',#36751,'mechanical');
#36759=PRODUCT('Feed Track Steel Guide Channel',
'Feed Track Steel Guide Channel',$,(#36752));
#36770=PRESENTATION_STYLE_ASSIGNMENT((#36777));
#36777=SURFACE_STYLE_USAGE(.BOTH.,#36784);
#36784=SURFACE_SIDE_STYLE('',(#36791));
#36791=SURFACE_STYLE_FILL_AREA(#36798);
#36798=FILL_AREA_STYLE('Opaque(169,212,242)',(#36805));
#36805=FILL_AREA_STYLE_COLOUR('Opaque(169,212,242)',#36812);
#36812=COLOUR_RGB('Opaque(169,212,242)',0.662745098039216,0.831372549019608,
0.949019607843137);
ENDSEC;
END-ISO-10303-21;
